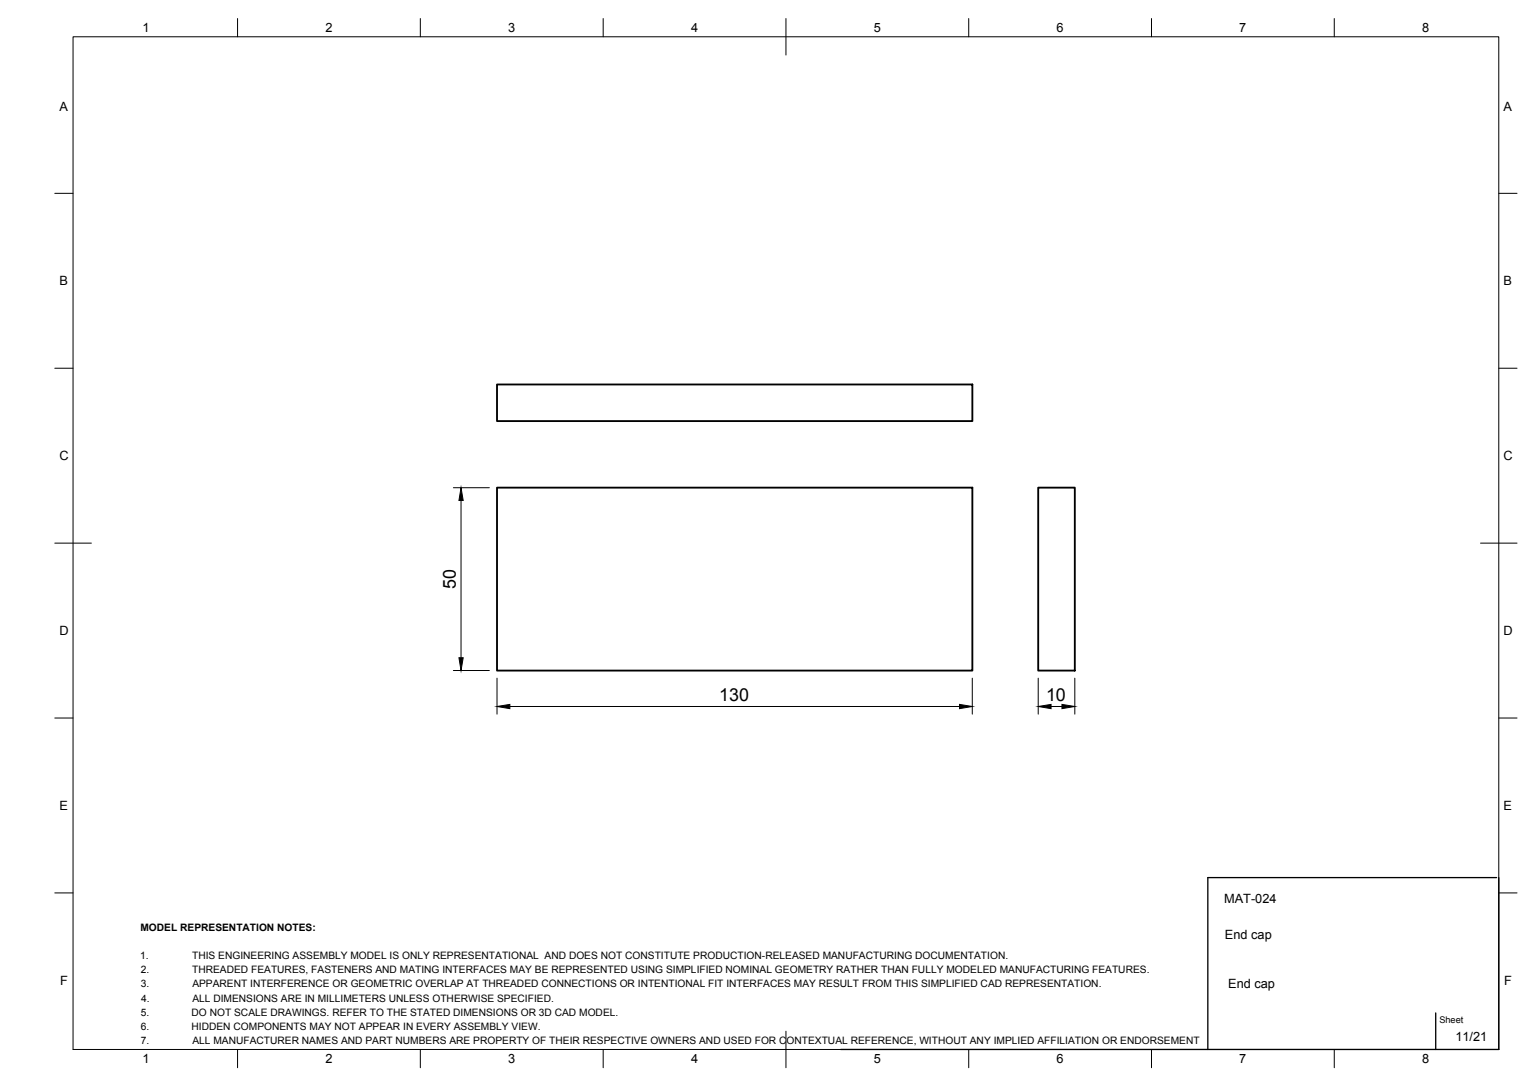
ISO-10303-21;
HEADER;
/* Generated by software containing ST-Developer
 * from STEP Tools, Inc. (www.steptools.com) 
 */

FILE_DESCRIPTION(
/* description */ ('STEP AP214'),
/* implementation_level */ '2;1');

FILE_NAME(
/* name */ 'End Cap.step',
/* time_stamp */ '2026-11-14T06:34:07-08:00',
/* author */ (''),
/* organization */ (''),
/* preprocessor_version */ 'ST-DEVELOPER v20.2',
/* originating_system */ 'Autodesk Translation Framework v15.17.0.0',
/* authorisation */ '');

FILE_SCHEMA (('AUTOMOTIVE_DESIGN { 1 0 10303 214 3 1 1 }'));
ENDSEC;

DATA;
#10=MECHANICAL_DESIGN_GEOMETRIC_PRESENTATION_REPRESENTATION('',(#7319),#310623);
#7234=SHAPE_REPRESENTATION_RELATIONSHIP('SRR','None',#310907,#7251);
#7251=ADVANCED_BREP_SHAPE_REPRESENTATION('',(#7386),#310616);
#7319=STYLED_ITEM('',(#311004),#7386);
#7386=MANIFOLD_SOLID_BREP('Body1',#93770);
#8626=PLANE('',#104555);
#8627=PLANE('',#104556);
#8628=PLANE('',#104557);
#8629=PLANE('',#104558);
#8630=PLANE('',#104559);
#8631=PLANE('',#104560);
#14237=FACE_OUTER_BOUND('',#20261,.T.);
#14238=FACE_OUTER_BOUND('',#20262,.T.);
#14239=FACE_OUTER_BOUND('',#20263,.T.);
#14240=FACE_OUTER_BOUND('',#20264,.T.);
#14241=FACE_OUTER_BOUND('',#20265,.T.);
#14242=FACE_OUTER_BOUND('',#20266,.T.);
#20261=EDGE_LOOP('',(#84791,#84792,#84793,#84794));
#20262=EDGE_LOOP('',(#84795,#84796,#84797,#84798));
#20263=EDGE_LOOP('',(#84799,#84800,#84801,#84802));
#20264=EDGE_LOOP('',(#84803,#84804,#84805,#84806));
#20265=EDGE_LOOP('',(#84807,#84808,#84809,#84810));
#20266=EDGE_LOOP('',(#84811,#84812,#84813,#84814));
#24628=LINE('',#302787,#28975);
#24629=LINE('',#302789,#28976);
#24630=LINE('',#302791,#28977);
#24631=LINE('',#302792,#28978);
#24632=LINE('',#302795,#28979);
#24633=LINE('',#302797,#28980);
#24634=LINE('',#302798,#28981);
#24635=LINE('',#302801,#28982);
#24636=LINE('',#302803,#28983);
#24637=LINE('',#302804,#28984);
#24638=LINE('',#302806,#28985);
#24639=LINE('',#302807,#28986);
#28975=VECTOR('',#130197,1000.);
#28976=VECTOR('',#130198,1000.);
#28977=VECTOR('',#130199,1000.);
#28978=VECTOR('',#130200,1000.);
#28979=VECTOR('',#130203,1000.);
#28980=VECTOR('',#130204,1000.);
#28981=VECTOR('',#130205,1000.);
#28982=VECTOR('',#130208,1000.);
#28983=VECTOR('',#130209,1000.);
#28984=VECTOR('',#130210,1000.);
#28985=VECTOR('',#130213,1000.);
#28986=VECTOR('',#130214,1000.);
#43298=VERTEX_POINT('',#302785);
#43299=VERTEX_POINT('',#302786);
#43300=VERTEX_POINT('',#302788);
#43301=VERTEX_POINT('',#302790);
#43302=VERTEX_POINT('',#302794);
#43303=VERTEX_POINT('',#302796);
#43304=VERTEX_POINT('',#302800);
#43305=VERTEX_POINT('',#302802);
#57175=EDGE_CURVE('',#43298,#43299,#24628,.T.);
#57176=EDGE_CURVE('',#43300,#43299,#24629,.T.);
#57177=EDGE_CURVE('',#43301,#43300,#24630,.T.);
#57178=EDGE_CURVE('',#43301,#43298,#24631,.T.);
#57179=EDGE_CURVE('',#43299,#43302,#24632,.T.);
#57180=EDGE_CURVE('',#43303,#43302,#24633,.T.);
#57181=EDGE_CURVE('',#43300,#43303,#24634,.T.);
#57182=EDGE_CURVE('',#43302,#43304,#24635,.T.);
#57183=EDGE_CURVE('',#43305,#43304,#24636,.T.);
#57184=EDGE_CURVE('',#43303,#43305,#24637,.T.);
#57185=EDGE_CURVE('',#43304,#43298,#24638,.T.);
#57186=EDGE_CURVE('',#43305,#43301,#24639,.T.);
#84791=ORIENTED_EDGE('',*,*,#57175,.T.);
#84792=ORIENTED_EDGE('',*,*,#57176,.F.);
#84793=ORIENTED_EDGE('',*,*,#57177,.F.);
#84794=ORIENTED_EDGE('',*,*,#57178,.T.);
#84795=ORIENTED_EDGE('',*,*,#57179,.T.);
#84796=ORIENTED_EDGE('',*,*,#57180,.F.);
#84797=ORIENTED_EDGE('',*,*,#57181,.F.);
#84798=ORIENTED_EDGE('',*,*,#57176,.T.);
#84799=ORIENTED_EDGE('',*,*,#57182,.T.);
#84800=ORIENTED_EDGE('',*,*,#57183,.F.);
#84801=ORIENTED_EDGE('',*,*,#57184,.F.);
#84802=ORIENTED_EDGE('',*,*,#57180,.T.);
#84803=ORIENTED_EDGE('',*,*,#57185,.T.);
#84804=ORIENTED_EDGE('',*,*,#57178,.F.);
#84805=ORIENTED_EDGE('',*,*,#57186,.F.);
#84806=ORIENTED_EDGE('',*,*,#57183,.T.);
#84807=ORIENTED_EDGE('',*,*,#57177,.T.);
#84808=ORIENTED_EDGE('',*,*,#57181,.T.);
#84809=ORIENTED_EDGE('',*,*,#57184,.T.);
#84810=ORIENTED_EDGE('',*,*,#57186,.T.);
#84811=ORIENTED_EDGE('',*,*,#57175,.F.);
#84812=ORIENTED_EDGE('',*,*,#57185,.F.);
#84813=ORIENTED_EDGE('',*,*,#57182,.F.);
#84814=ORIENTED_EDGE('',*,*,#57179,.F.);
#93516=ADVANCED_FACE('',(#14237),#8626,.F.);
#93517=ADVANCED_FACE('',(#14238),#8627,.F.);
#93518=ADVANCED_FACE('',(#14239),#8628,.F.);
#93519=ADVANCED_FACE('',(#14240),#8629,.F.);
#93520=ADVANCED_FACE('',(#14241),#8630,.F.);
#93521=ADVANCED_FACE('',(#14242),#8631,.T.);
#93770=CLOSED_SHELL('',(#93516,#93517,#93518,#93519,#93520,#93521));
#104554=AXIS2_PLACEMENT_3D('',#302783,#130193,#130194);
#104555=AXIS2_PLACEMENT_3D('',#302784,#130195,#130196);
#104556=AXIS2_PLACEMENT_3D('',#302793,#130201,#130202);
#104557=AXIS2_PLACEMENT_3D('',#302799,#130206,#130207);
#104558=AXIS2_PLACEMENT_3D('',#302805,#130211,#130212);
#104559=AXIS2_PLACEMENT_3D('',#302808,#130215,#130216);
#104560=AXIS2_PLACEMENT_3D('',#302809,#130217,#130218);
#130193=DIRECTION('axis',(0.,0.,1.));
#130194=DIRECTION('refdir',(1.,0.,0.));
#130195=DIRECTION('center_axis',(-1.,0.,0.));
#130196=DIRECTION('ref_axis',(0.,0.,1.));
#130197=DIRECTION('',(0.,1.,0.));
#130198=DIRECTION('',(0.,0.,-1.));
#130199=DIRECTION('',(0.,1.,0.));
#130200=DIRECTION('',(0.,0.,-1.));
#130201=DIRECTION('center_axis',(0.,-1.,0.));
#130202=DIRECTION('ref_axis',(0.,0.,-1.));
#130203=DIRECTION('',(-1.,0.,0.));
#130204=DIRECTION('',(0.,0.,-1.));
#130205=DIRECTION('',(-1.,0.,0.));
#130206=DIRECTION('center_axis',(1.,4.2700885562506E-16,0.));
#130207=DIRECTION('ref_axis',(-4.2700885562506E-16,1.,0.));
#130208=DIRECTION('',(4.2700885562506E-16,-1.,0.));
#130209=DIRECTION('',(0.,0.,-1.));
#130210=DIRECTION('',(4.2700885562506E-16,-1.,0.));
#130211=DIRECTION('center_axis',(-5.55111512312578E-16,1.,0.));
#130212=DIRECTION('ref_axis',(-1.,-5.55111512312578E-16,0.));
#130213=DIRECTION('',(1.,5.55111512312578E-16,0.));
#130214=DIRECTION('',(1.,5.55111512312578E-16,0.));
#130215=DIRECTION('center_axis',(0.,0.,-1.));
#130216=DIRECTION('ref_axis',(-1.,0.,0.));
#130217=DIRECTION('center_axis',(0.,0.,-1.));
#130218=DIRECTION('ref_axis',(-1.,0.,0.));
#302783=CARTESIAN_POINT('',(0.,0.,0.));
#302784=CARTESIAN_POINT('Origin',(346.089749425718,367.316749888869,10.));
#302785=CARTESIAN_POINT('',(346.089749425718,237.316749888869,0.));
#302786=CARTESIAN_POINT('',(346.089749425718,367.316749888869,0.));
#302787=CARTESIAN_POINT('',(346.089749425718,367.316749888869,0.));
#302788=CARTESIAN_POINT('',(346.089749425718,367.316749888869,10.));
#302789=CARTESIAN_POINT('',(346.089749425718,367.316749888869,10.));
#302790=CARTESIAN_POINT('',(346.089749425718,237.316749888869,10.));
#302791=CARTESIAN_POINT('',(346.089749425718,367.316749888869,10.));
#302792=CARTESIAN_POINT('',(346.089749425718,237.316749888869,10.));
#302793=CARTESIAN_POINT('Origin',(346.089749425718,367.316749888869,10.));
#302794=CARTESIAN_POINT('',(296.089749425718,367.316749888869,0.));
#302795=CARTESIAN_POINT('',(346.089749425718,367.316749888869,0.));
#302796=CARTESIAN_POINT('',(296.089749425718,367.316749888869,10.));
#302797=CARTESIAN_POINT('',(296.089749425718,367.316749888869,10.));
#302798=CARTESIAN_POINT('',(346.089749425718,367.316749888869,10.));
#302799=CARTESIAN_POINT('Origin',(296.089749425718,367.316749888869,10.));
#302800=CARTESIAN_POINT('',(296.089749425718,237.316749888869,0.));
#302801=CARTESIAN_POINT('',(296.089749425718,367.316749888869,0.));
#302802=CARTESIAN_POINT('',(296.089749425718,237.316749888869,10.));
#302803=CARTESIAN_POINT('',(296.089749425718,237.316749888869,10.));
#302804=CARTESIAN_POINT('',(296.089749425718,367.316749888869,10.));
#302805=CARTESIAN_POINT('Origin',(346.089749425718,237.316749888869,10.));
#302806=CARTESIAN_POINT('',(346.089749425718,237.316749888869,0.));
#302807=CARTESIAN_POINT('',(346.089749425718,237.316749888869,10.));
#302808=CARTESIAN_POINT('Origin',(0.,0.,10.));
#302809=CARTESIAN_POINT('Origin',(0.,0.,0.));
#310594=UNCERTAINTY_MEASURE_WITH_UNIT(LENGTH_MEASURE(0.01),#310624,
'DISTANCE_ACCURACY_VALUE',
'Maximum model space distance between geometric entities at asserted c
onnectivities');
#310601=UNCERTAINTY_MEASURE_WITH_UNIT(LENGTH_MEASURE(0.01),#310624,
'DISTANCE_ACCURACY_VALUE',
'Maximum model space distance between geometric entities at asserted c
onnectivities');
#310616=(
GEOMETRIC_REPRESENTATION_CONTEXT(3)
GLOBAL_UNCERTAINTY_ASSIGNED_CONTEXT((#310594))
GLOBAL_UNIT_ASSIGNED_CONTEXT((#310624,#310626,#310627))
REPRESENTATION_CONTEXT('','3D')
);
#310623=(
GEOMETRIC_REPRESENTATION_CONTEXT(3)
GLOBAL_UNCERTAINTY_ASSIGNED_CONTEXT((#310601))
GLOBAL_UNIT_ASSIGNED_CONTEXT((#310624,#310626,#310627))
REPRESENTATION_CONTEXT('','3D')
);
#310624=(
LENGTH_UNIT()
NAMED_UNIT(*)
SI_UNIT(.MILLI.,.METRE.)
);
#310626=(
NAMED_UNIT(*)
PLANE_ANGLE_UNIT()
SI_UNIT($,.RADIAN.)
);
#310627=(
NAMED_UNIT(*)
SI_UNIT($,.STERADIAN.)
SOLID_ANGLE_UNIT()
);
#310642=SHAPE_DEFINITION_REPRESENTATION(#310801,#310907);
#310801=PRODUCT_DEFINITION_SHAPE('',$,#310929);
#310907=SHAPE_REPRESENTATION('',(#104554),#310616);
#310914=PRODUCT_DEFINITION_CONTEXT('part definition',#310979,'design');
#310929=PRODUCT_DEFINITION('End cap','End Cap',#310950,#310914);
#310950=PRODUCT_DEFINITION_FORMATION('',$,#310995);
#310979=APPLICATION_CONTEXT(
'Core Data for Automotive Mechanical Design Process');
#310980=PRODUCT_CONTEXT('part definition',#310979,'mechanical');
#310995=PRODUCT('End cap','End Cap','End cap',(#310980));
#311004=PRESENTATION_STYLE_ASSIGNMENT((#311011));
#311011=SURFACE_STYLE_USAGE(.BOTH.,#311018);
#311018=SURFACE_SIDE_STYLE('',(#311025));
#311025=SURFACE_STYLE_FILL_AREA(#311032);
#311032=FILL_AREA_STYLE('Opaque(227,224,212)',(#311039));
#311039=FILL_AREA_STYLE_COLOUR('Opaque(227,224,212)',#311046);
#311046=COLOUR_RGB('Opaque(227,224,212)',0.890196078431372,0.87843137254902,
0.831372549019608);
ENDSEC;
END-ISO-10303-21;
